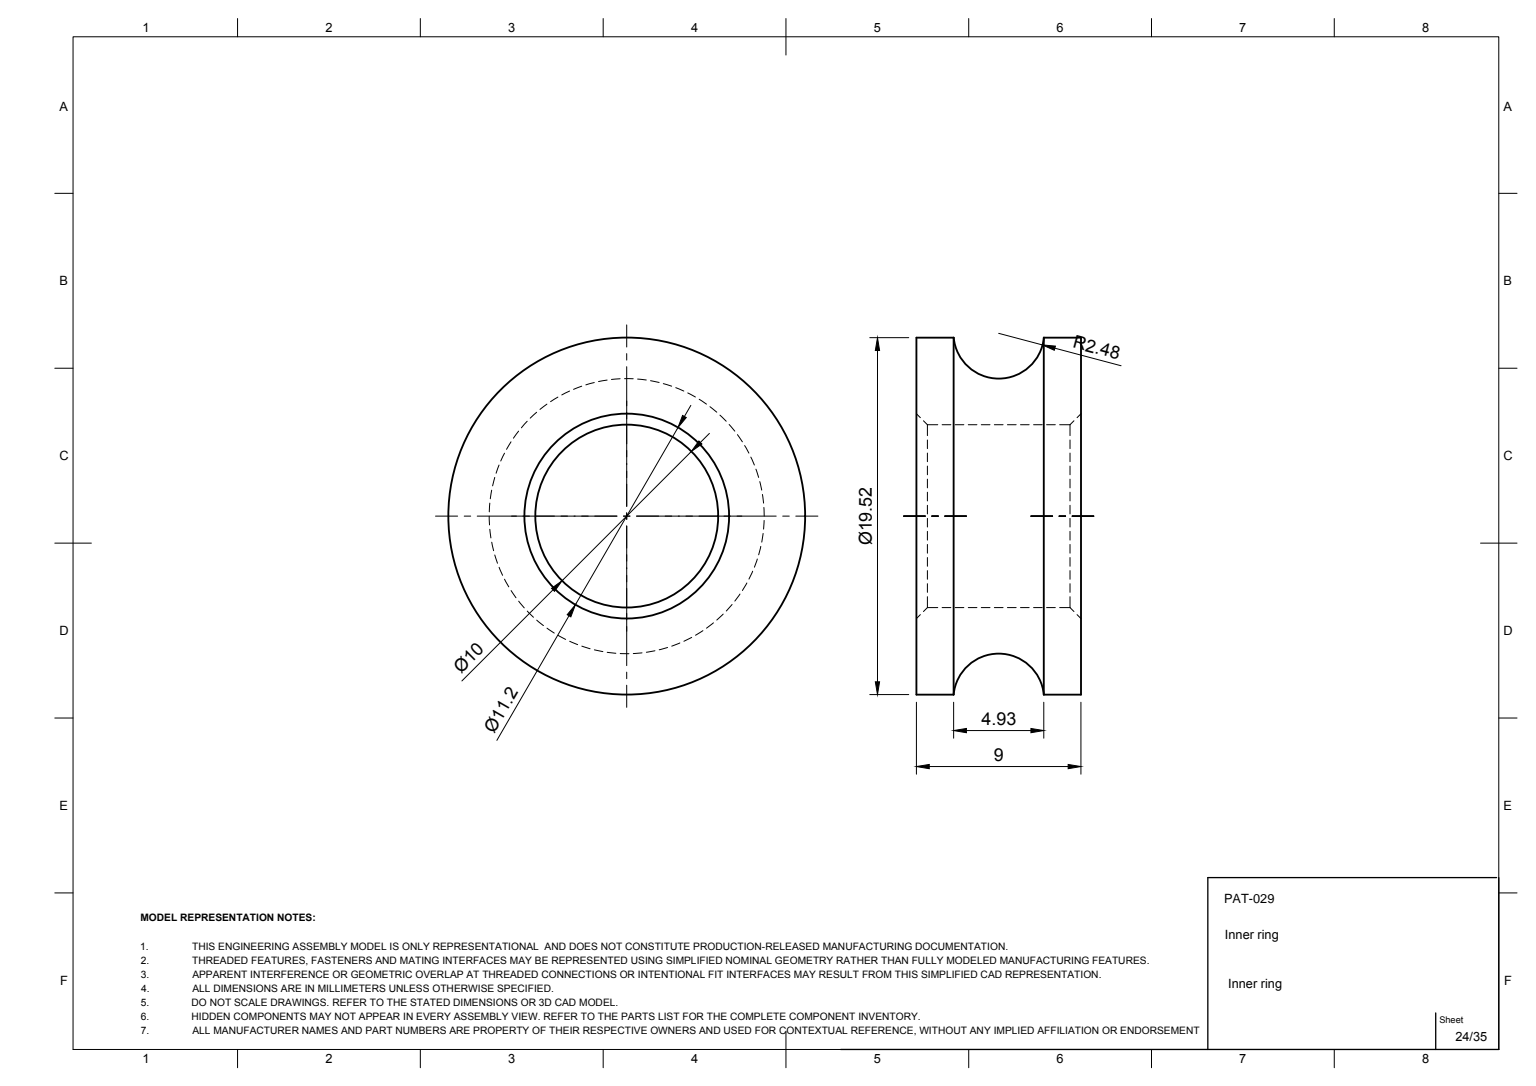
ISO-10303-21;
HEADER;
/* Generated by software containing ST-Developer
 * from STEP Tools, Inc. (www.steptools.com) 
 */

FILE_DESCRIPTION(
/* description */ ('Door-style hinge test fixture with detent'),
/* implementation_level */ '2;1');

FILE_NAME(
/* name */ 'Inner ring.step',
/* time_stamp */ '2026-10-28T03:24:57-07:00',
/* author */ (''),
/* organization */ (''),
/* preprocessor_version */ 'ST-DEVELOPER v20.2',
/* originating_system */ 'Autodesk Translation Framework v15.17.0.0',
/* authorisation */ '');

FILE_SCHEMA (('AUTOMOTIVE_DESIGN { 1 0 10303 214 3 1 1 }'));
ENDSEC;

DATA;
#10=MECHANICAL_DESIGN_GEOMETRIC_PRESENTATION_REPRESENTATION('',(#342),#9813);
#199=TOROIDAL_SURFACE('',#5444,1.,0.247676);
#204=CONICAL_SURFACE('',#5455,0.53,0.785398163397448);
#205=CONICAL_SURFACE('',#5462,0.53,0.785398163397448);
#279=SHAPE_REPRESENTATION_RELATIONSHIP('SRR','None',#9957,#310);
#310=ADVANCED_BREP_SHAPE_REPRESENTATION('',(#381),#9800);
#342=STYLED_ITEM('',(#10183),#381);
#381=MANIFOLD_SOLID_BREP('Body1',#4774);
#468=FACE_BOUND('',#1184,.T.);
#469=FACE_BOUND('',#1187,.T.);
#605=PLANE('',#5457);
#606=PLANE('',#5460);
#825=FACE_OUTER_BOUND('',#1179,.T.);
#826=FACE_OUTER_BOUND('',#1180,.T.);
#827=FACE_OUTER_BOUND('',#1181,.T.);
#828=FACE_OUTER_BOUND('',#1182,.T.);
#829=FACE_OUTER_BOUND('',#1183,.T.);
#830=FACE_OUTER_BOUND('',#1185,.T.);
#831=FACE_OUTER_BOUND('',#1186,.T.);
#832=FACE_OUTER_BOUND('',#1188,.T.);
#1179=EDGE_LOOP('',(#3899,#3900,#3901,#3902,#3903,#3904));
#1180=EDGE_LOOP('',(#3905,#3906,#3907,#3908,#3909));
#1181=EDGE_LOOP('',(#3910,#3911,#3912,#3913));
#1182=EDGE_LOOP('',(#3914,#3915,#3916,#3917));
#1183=EDGE_LOOP('',(#3918));
#1184=EDGE_LOOP('',(#3919));
#1185=EDGE_LOOP('',(#3920,#3921,#3922,#3923,#3924));
#1186=EDGE_LOOP('',(#3925));
#1187=EDGE_LOOP('',(#3926));
#1188=EDGE_LOOP('',(#3927,#3928,#3929,#3930));
#1557=LINE('',#8784,#1877);
#1558=LINE('',#8790,#1878);
#1559=LINE('',#8794,#1879);
#1560=LINE('',#8800,#1880);
#1561=LINE('',#8805,#1881);
#1877=VECTOR('',#6600,0.976185);
#1878=VECTOR('',#6607,0.5);
#1879=VECTOR('',#6612,0.53);
#1880=VECTOR('',#6621,0.976185);
#1881=VECTOR('',#6628,0.53);
#2096=CIRCLE('',#5445,0.976185);
#2097=CIRCLE('',#5446,0.976185);
#2098=CIRCLE('',#5447,0.247676);
#2099=CIRCLE('',#5448,0.976185);
#2100=CIRCLE('',#5449,0.976185);
#2101=CIRCLE('',#5451,0.976185);
#2102=CIRCLE('',#5453,0.5);
#2103=CIRCLE('',#5454,0.5);
#2104=CIRCLE('',#5456,0.56);
#2105=CIRCLE('',#5459,0.976185);
#2106=CIRCLE('',#5461,0.56);
#2452=VERTEX_POINT('',#8773);
#2453=VERTEX_POINT('',#8774);
#2454=VERTEX_POINT('',#8777);
#2455=VERTEX_POINT('',#8779);
#2456=VERTEX_POINT('',#8783);
#2457=VERTEX_POINT('',#8787);
#2458=VERTEX_POINT('',#8789);
#2459=VERTEX_POINT('',#8793);
#2460=VERTEX_POINT('',#8798);
#2461=VERTEX_POINT('',#8802);
#2966=EDGE_CURVE('',#2452,#2453,#2096,.T.);
#2967=EDGE_CURVE('',#2453,#2452,#2097,.T.);
#2968=EDGE_CURVE('',#2453,#2454,#2098,.T.);
#2969=EDGE_CURVE('',#2455,#2454,#2099,.T.);
#2970=EDGE_CURVE('',#2454,#2455,#2100,.T.);
#2971=EDGE_CURVE('',#2455,#2456,#1557,.T.);
#2972=EDGE_CURVE('',#2456,#2456,#2101,.T.);
#2973=EDGE_CURVE('',#2457,#2457,#2102,.T.);
#2974=EDGE_CURVE('',#2457,#2458,#1558,.T.);
#2975=EDGE_CURVE('',#2458,#2458,#2103,.T.);
#2976=EDGE_CURVE('',#2458,#2459,#1559,.T.);
#2977=EDGE_CURVE('',#2459,#2459,#2104,.T.);
#2978=EDGE_CURVE('',#2460,#2460,#2105,.T.);
#2979=EDGE_CURVE('',#2460,#2452,#1560,.T.);
#2980=EDGE_CURVE('',#2461,#2461,#2106,.T.);
#2981=EDGE_CURVE('',#2461,#2457,#1561,.T.);
#3899=ORIENTED_EDGE('',*,*,#2966,.F.);
#3900=ORIENTED_EDGE('',*,*,#2967,.F.);
#3901=ORIENTED_EDGE('',*,*,#2968,.T.);
#3902=ORIENTED_EDGE('',*,*,#2969,.F.);
#3903=ORIENTED_EDGE('',*,*,#2970,.F.);
#3904=ORIENTED_EDGE('',*,*,#2968,.F.);
#3905=ORIENTED_EDGE('',*,*,#2969,.T.);
#3906=ORIENTED_EDGE('',*,*,#2970,.T.);
#3907=ORIENTED_EDGE('',*,*,#2971,.T.);
#3908=ORIENTED_EDGE('',*,*,#2972,.T.);
#3909=ORIENTED_EDGE('',*,*,#2971,.F.);
#3910=ORIENTED_EDGE('',*,*,#2973,.T.);
#3911=ORIENTED_EDGE('',*,*,#2974,.T.);
#3912=ORIENTED_EDGE('',*,*,#2975,.F.);
#3913=ORIENTED_EDGE('',*,*,#2974,.F.);
#3914=ORIENTED_EDGE('',*,*,#2975,.T.);
#3915=ORIENTED_EDGE('',*,*,#2976,.T.);
#3916=ORIENTED_EDGE('',*,*,#2977,.F.);
#3917=ORIENTED_EDGE('',*,*,#2976,.F.);
#3918=ORIENTED_EDGE('',*,*,#2972,.F.);
#3919=ORIENTED_EDGE('',*,*,#2977,.T.);
#3920=ORIENTED_EDGE('',*,*,#2978,.F.);
#3921=ORIENTED_EDGE('',*,*,#2979,.T.);
#3922=ORIENTED_EDGE('',*,*,#2966,.T.);
#3923=ORIENTED_EDGE('',*,*,#2967,.T.);
#3924=ORIENTED_EDGE('',*,*,#2979,.F.);
#3925=ORIENTED_EDGE('',*,*,#2978,.T.);
#3926=ORIENTED_EDGE('',*,*,#2980,.F.);
#3927=ORIENTED_EDGE('',*,*,#2980,.T.);
#3928=ORIENTED_EDGE('',*,*,#2981,.T.);
#3929=ORIENTED_EDGE('',*,*,#2973,.F.);
#3930=ORIENTED_EDGE('',*,*,#2981,.F.);
#4433=CYLINDRICAL_SURFACE('',#5450,0.976185);
#4434=CYLINDRICAL_SURFACE('',#5452,0.5);
#4435=CYLINDRICAL_SURFACE('',#5458,0.976185);
#4630=ADVANCED_FACE('',(#825),#199,.F.);
#4631=ADVANCED_FACE('',(#826),#4433,.T.);
#4632=ADVANCED_FACE('',(#827),#4434,.F.);
#4633=ADVANCED_FACE('',(#828),#204,.F.);
#4634=ADVANCED_FACE('',(#829,#468),#605,.T.);
#4635=ADVANCED_FACE('',(#830),#4435,.T.);
#4636=ADVANCED_FACE('',(#831,#469),#606,.T.);
#4637=ADVANCED_FACE('',(#832),#205,.F.);
#4774=CLOSED_SHELL('',(#4630,#4631,#4632,#4633,#4634,#4635,#4636,#4637));
#5443=AXIS2_PLACEMENT_3D('',#8771,#6584,#6585);
#5444=AXIS2_PLACEMENT_3D('',#8772,#6586,#6587);
#5445=AXIS2_PLACEMENT_3D('',#8775,#6588,#6589);
#5446=AXIS2_PLACEMENT_3D('',#8776,#6590,#6591);
#5447=AXIS2_PLACEMENT_3D('',#8778,#6592,#6593);
#5448=AXIS2_PLACEMENT_3D('',#8780,#6594,#6595);
#5449=AXIS2_PLACEMENT_3D('',#8781,#6596,#6597);
#5450=AXIS2_PLACEMENT_3D('',#8782,#6598,#6599);
#5451=AXIS2_PLACEMENT_3D('',#8785,#6601,#6602);
#5452=AXIS2_PLACEMENT_3D('',#8786,#6603,#6604);
#5453=AXIS2_PLACEMENT_3D('',#8788,#6605,#6606);
#5454=AXIS2_PLACEMENT_3D('',#8791,#6608,#6609);
#5455=AXIS2_PLACEMENT_3D('',#8792,#6610,#6611);
#5456=AXIS2_PLACEMENT_3D('',#8795,#6613,#6614);
#5457=AXIS2_PLACEMENT_3D('',#8796,#6615,#6616);
#5458=AXIS2_PLACEMENT_3D('',#8797,#6617,#6618);
#5459=AXIS2_PLACEMENT_3D('',#8799,#6619,#6620);
#5460=AXIS2_PLACEMENT_3D('',#8801,#6622,#6623);
#5461=AXIS2_PLACEMENT_3D('',#8803,#6624,#6625);
#5462=AXIS2_PLACEMENT_3D('',#8804,#6626,#6627);
#6584=DIRECTION('axis',(0.,0.,1.));
#6585=DIRECTION('refdir',(1.,0.,0.));
#6586=DIRECTION('center_axis',(0.,-1.,0.));
#6587=DIRECTION('ref_axis',(0.,0.,-1.));
#6588=DIRECTION('center_axis',(0.,-1.,0.));
#6589=DIRECTION('ref_axis',(1.,0.,0.));
#6590=DIRECTION('center_axis',(0.,-1.,0.));
#6591=DIRECTION('ref_axis',(1.,0.,0.));
#6592=DIRECTION('center_axis',(1.,0.,1.22464679914735E-16));
#6593=DIRECTION('ref_axis',(-1.22464679914735E-16,0.,1.));
#6594=DIRECTION('center_axis',(0.,1.,0.));
#6595=DIRECTION('ref_axis',(1.,0.,0.));
#6596=DIRECTION('center_axis',(0.,1.,0.));
#6597=DIRECTION('ref_axis',(1.,0.,0.));
#6598=DIRECTION('center_axis',(0.,-1.,0.));
#6599=DIRECTION('ref_axis',(1.,0.,0.));
#6600=DIRECTION('',(0.,1.,0.));
#6601=DIRECTION('center_axis',(0.,-1.,0.));
#6602=DIRECTION('ref_axis',(1.,0.,0.));
#6603=DIRECTION('center_axis',(0.,-1.,0.));
#6604=DIRECTION('ref_axis',(1.,0.,0.));
#6605=DIRECTION('center_axis',(0.,-1.,0.));
#6606=DIRECTION('ref_axis',(1.,0.,0.));
#6607=DIRECTION('',(0.,1.,0.));
#6608=DIRECTION('center_axis',(0.,-1.,0.));
#6609=DIRECTION('ref_axis',(1.,0.,0.));
#6610=DIRECTION('center_axis',(0.,1.,0.));
#6611=DIRECTION('ref_axis',(1.,0.,0.));
#6612=DIRECTION('',(-0.707106781186547,0.707106781186548,-8.65956056235493E-17));
#6613=DIRECTION('center_axis',(0.,-1.,0.));
#6614=DIRECTION('ref_axis',(1.,0.,0.));
#6615=DIRECTION('center_axis',(0.,1.,0.));
#6616=DIRECTION('ref_axis',(0.,0.,1.));
#6617=DIRECTION('center_axis',(0.,-1.,0.));
#6618=DIRECTION('ref_axis',(1.,0.,0.));
#6619=DIRECTION('center_axis',(0.,-1.,0.));
#6620=DIRECTION('ref_axis',(1.,0.,0.));
#6621=DIRECTION('',(0.,1.,0.));
#6622=DIRECTION('center_axis',(0.,-1.,0.));
#6623=DIRECTION('ref_axis',(0.,0.,-1.));
#6624=DIRECTION('center_axis',(0.,-1.,0.));
#6625=DIRECTION('ref_axis',(1.,0.,0.));
#6626=DIRECTION('center_axis',(0.,-1.,0.));
#6627=DIRECTION('ref_axis',(1.,0.,0.));
#6628=DIRECTION('',(0.707106781186547,0.707106781186548,8.65956056235493E-17));
#8771=CARTESIAN_POINT('',(0.,0.,0.));
#8772=CARTESIAN_POINT('Origin',(0.,0.,0.));
#8773=CARTESIAN_POINT('',(-0.976185,-0.246528389340863,-1.19548183562566E-16));
#8774=CARTESIAN_POINT('',(-1.19548183562566E-16,-0.246528389340863,0.976185));
#8775=CARTESIAN_POINT('Origin',(0.,-0.246528389340863,0.));
#8776=CARTESIAN_POINT('Origin',(0.,-0.246528389340863,0.));
#8777=CARTESIAN_POINT('',(-1.19548183562566E-16,0.246528389340863,0.976185));
#8778=CARTESIAN_POINT('Origin',(-1.22464679914735E-16,0.,1.));
#8779=CARTESIAN_POINT('',(-0.976185,0.246528389340863,1.19548183562566E-16));
#8780=CARTESIAN_POINT('Origin',(0.,0.246528389340863,0.));
#8781=CARTESIAN_POINT('Origin',(0.,0.246528389340863,0.));
#8782=CARTESIAN_POINT('Origin',(0.,0.,0.));
#8783=CARTESIAN_POINT('',(-0.976185,0.45,-1.19548183562566E-16));
#8784=CARTESIAN_POINT('',(-0.976185,0.,-1.19548183562566E-16));
#8785=CARTESIAN_POINT('Origin',(0.,0.45,0.));
#8786=CARTESIAN_POINT('Origin',(0.,0.,0.));
#8787=CARTESIAN_POINT('',(-0.5,-0.39,-6.12323399573677E-17));
#8788=CARTESIAN_POINT('Origin',(0.,-0.39,0.));
#8789=CARTESIAN_POINT('',(-0.5,0.39,-6.12323399573677E-17));
#8790=CARTESIAN_POINT('',(-0.5,0.,-6.12323399573677E-17));
#8791=CARTESIAN_POINT('Origin',(0.,0.39,0.));
#8792=CARTESIAN_POINT('Origin',(0.,0.42,0.));
#8793=CARTESIAN_POINT('',(-0.56,0.45,-6.85802207522518E-17));
#8794=CARTESIAN_POINT('',(-0.53,0.42,-6.49062803548097E-17));
#8795=CARTESIAN_POINT('Origin',(0.,0.45,0.));
#8796=CARTESIAN_POINT('Origin',(0.976185,0.45,0.));
#8797=CARTESIAN_POINT('Origin',(0.,0.,0.));
#8798=CARTESIAN_POINT('',(-0.976185,-0.45,-1.19548183562566E-16));
#8799=CARTESIAN_POINT('Origin',(0.,-0.45,0.));
#8800=CARTESIAN_POINT('',(-0.976185,0.,-1.19548183562566E-16));
#8801=CARTESIAN_POINT('Origin',(0.56,-0.45,0.));
#8802=CARTESIAN_POINT('',(-0.56,-0.45,-6.85802207522518E-17));
#8803=CARTESIAN_POINT('Origin',(0.,-0.45,0.));
#8804=CARTESIAN_POINT('Origin',(0.,-0.42,0.));
#8805=CARTESIAN_POINT('',(-0.53,-0.42,-6.49062803548097E-17));
#9764=UNCERTAINTY_MEASURE_WITH_UNIT(LENGTH_MEASURE(0.001),#9814,
'DISTANCE_ACCURACY_VALUE',
'Maximum model space distance between geometric entities at asserted c
onnectivities');
#9777=UNCERTAINTY_MEASURE_WITH_UNIT(LENGTH_MEASURE(0.001),#9814,
'DISTANCE_ACCURACY_VALUE',
'Maximum model space distance between geometric entities at asserted c
onnectivities');
#9800=(
GEOMETRIC_REPRESENTATION_CONTEXT(3)
GLOBAL_UNCERTAINTY_ASSIGNED_CONTEXT((#9764))
GLOBAL_UNIT_ASSIGNED_CONTEXT((#9814,#9816,#9817))
REPRESENTATION_CONTEXT('','3D')
);
#9813=(
GEOMETRIC_REPRESENTATION_CONTEXT(3)
GLOBAL_UNCERTAINTY_ASSIGNED_CONTEXT((#9777))
GLOBAL_UNIT_ASSIGNED_CONTEXT((#9814,#9816,#9817))
REPRESENTATION_CONTEXT('','3D')
);
#9814=(
LENGTH_UNIT()
NAMED_UNIT(*)
SI_UNIT(.CENTI.,.METRE.)
);
#9816=(
NAMED_UNIT(*)
PLANE_ANGLE_UNIT()
SI_UNIT($,.RADIAN.)
);
#9817=(
NAMED_UNIT(*)
SI_UNIT($,.STERADIAN.)
SOLID_ANGLE_UNIT()
);
#9840=SHAPE_DEFINITION_REPRESENTATION(#9875,#9957);
#9875=PRODUCT_DEFINITION_SHAPE('',$,#9993);
#9957=SHAPE_REPRESENTATION('',(#5443),#9800);
#9970=PRODUCT_DEFINITION_CONTEXT('part definition',#10077,'design');
#9993=PRODUCT_DEFINITION('Inner ring','Inner ring',#10028,#9970);
#10028=PRODUCT_DEFINITION_FORMATION('',$,#10101);
#10077=APPLICATION_CONTEXT(
'Core Data for Automotive Mechanical Design Process');
#10078=PRODUCT_CONTEXT('part definition',#10077,'mechanical');
#10101=PRODUCT('Inner ring','Inner ring','Inner ring',(#10078));
#10177=COLOUR_RGB('Grey',0.48,0.52,0.57);
#10178=FILL_AREA_STYLE_COLOUR('',#10177);
#10179=FILL_AREA_STYLE('',(#10178));
#10180=SURFACE_STYLE_FILL_AREA(#10179);
#10181=SURFACE_SIDE_STYLE('',(#10180));
#10182=SURFACE_STYLE_USAGE(.BOTH.,#10181);
#10183=PRESENTATION_STYLE_ASSIGNMENT((#10182));
ENDSEC;
END-ISO-10303-21;
